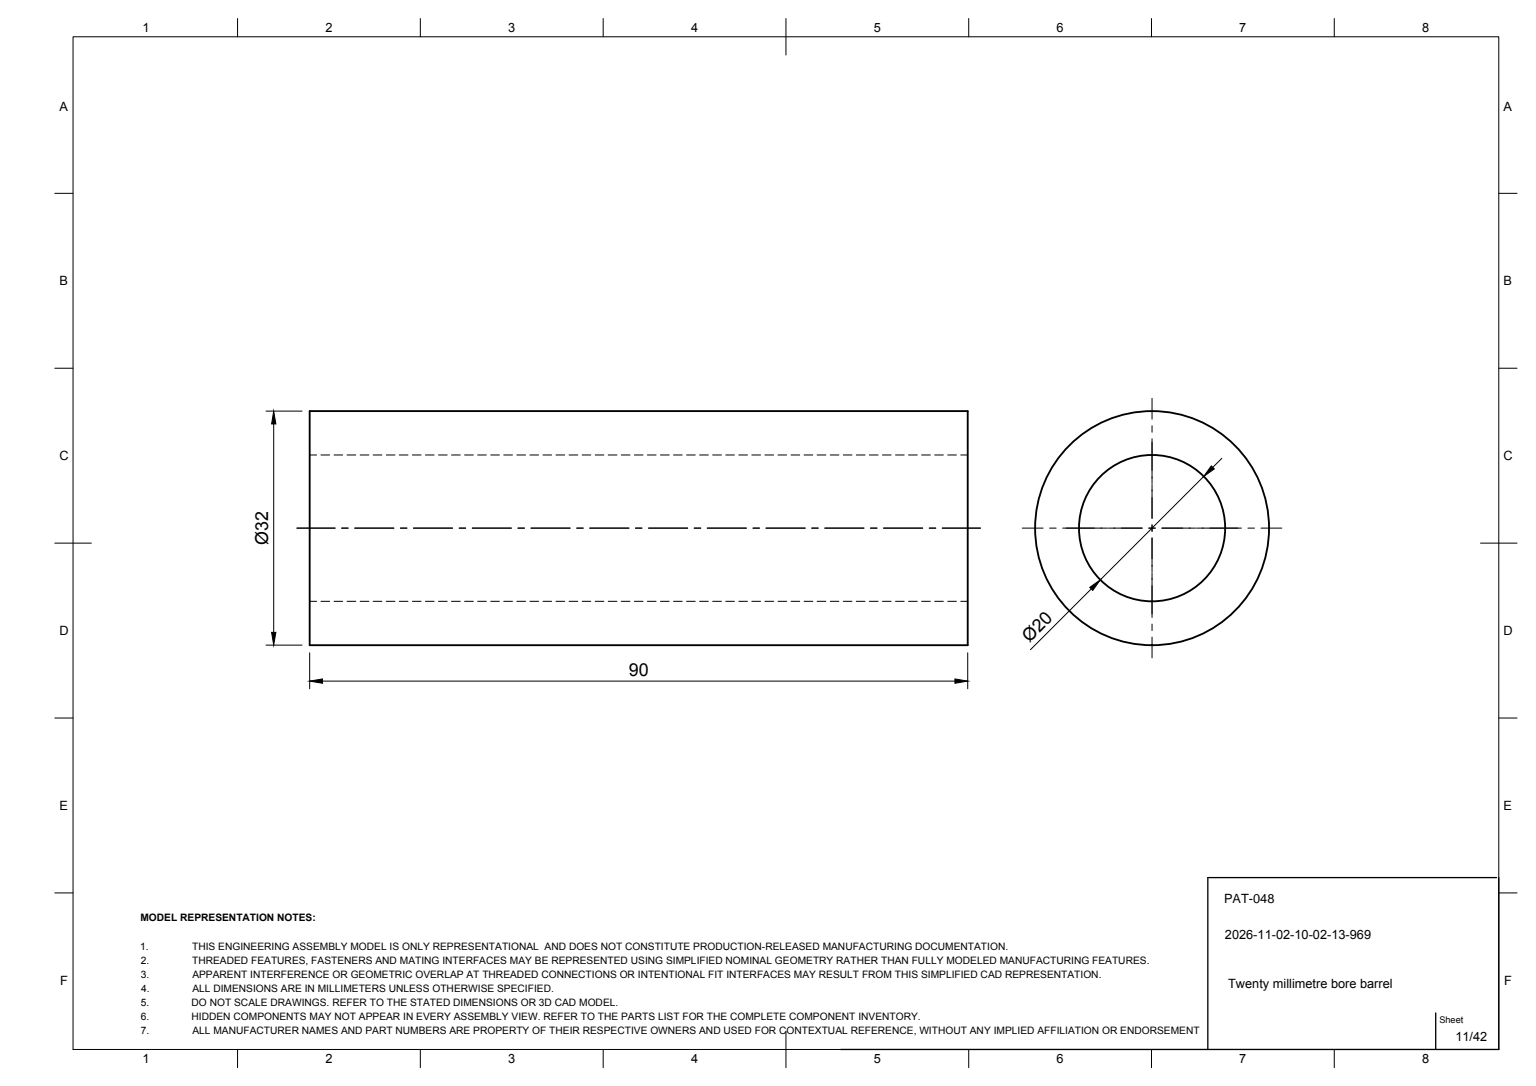
ISO-10303-21;
HEADER;
/* Generated by software containing ST-Developer
 * from STEP Tools, Inc. (www.steptools.com) 
 */

FILE_DESCRIPTION(
/* description */ ('Guided pneumatic stop gate'),
/* implementation_level */ '2;1');

FILE_NAME(
/* name */ 'Twenty millimetre bore barrel.step',
/* time_stamp */ '2026-10-27T21:43:45-07:00',
/* author */ (''),
/* organization */ (''),
/* preprocessor_version */ 'ST-DEVELOPER v20.2',
/* originating_system */ 'Autodesk Translation Framework v15.17.0.0',
/* authorisation */ '');

FILE_SCHEMA (('AUTOMOTIVE_DESIGN { 1 0 10303 214 3 1 1 }'));
ENDSEC;

DATA;
#10=MECHANICAL_DESIGN_GEOMETRIC_PRESENTATION_REPRESENTATION('',(#541),#14392);
#457=SHAPE_REPRESENTATION_RELATIONSHIP('SRR','None',#14591,#499);
#499=ADVANCED_BREP_SHAPE_REPRESENTATION('',(#583),#14353);
#541=STYLED_ITEM('',(#14884),#583);
#583=MANIFOLD_SOLID_BREP('Body1',#7881);
#663=FACE_BOUND('',#1777,.T.);
#664=FACE_BOUND('',#1779,.T.);
#921=PLANE('',#8642);
#922=PLANE('',#8643);
#1251=FACE_OUTER_BOUND('',#1774,.T.);
#1252=FACE_OUTER_BOUND('',#1775,.T.);
#1253=FACE_OUTER_BOUND('',#1776,.T.);
#1254=FACE_OUTER_BOUND('',#1778,.T.);
#1774=EDGE_LOOP('',(#5862,#5863,#5864,#5865));
#1775=EDGE_LOOP('',(#5866,#5867,#5868,#5869));
#1776=EDGE_LOOP('',(#5870));
#1777=EDGE_LOOP('',(#5871));
#1778=EDGE_LOOP('',(#5872));
#1779=EDGE_LOOP('',(#5873));
#2441=LINE('',#12509,#2986);
#2442=LINE('',#12515,#2987);
#2986=VECTOR('',#10052,1.);
#2987=VECTOR('',#10059,1.6);
#3464=CIRCLE('',#8637,1.);
#3465=CIRCLE('',#8638,1.);
#3466=CIRCLE('',#8640,1.6);
#3467=CIRCLE('',#8641,1.6);
#3907=VERTEX_POINT('',#12506);
#3908=VERTEX_POINT('',#12508);
#3909=VERTEX_POINT('',#12512);
#3910=VERTEX_POINT('',#12514);
#4629=EDGE_CURVE('',#3907,#3907,#3464,.T.);
#4630=EDGE_CURVE('',#3907,#3908,#2441,.T.);
#4631=EDGE_CURVE('',#3908,#3908,#3465,.T.);
#4632=EDGE_CURVE('',#3909,#3909,#3466,.T.);
#4633=EDGE_CURVE('',#3909,#3910,#2442,.T.);
#4634=EDGE_CURVE('',#3910,#3910,#3467,.T.);
#5862=ORIENTED_EDGE('',*,*,#4629,.F.);
#5863=ORIENTED_EDGE('',*,*,#4630,.T.);
#5864=ORIENTED_EDGE('',*,*,#4631,.T.);
#5865=ORIENTED_EDGE('',*,*,#4630,.F.);
#5866=ORIENTED_EDGE('',*,*,#4632,.F.);
#5867=ORIENTED_EDGE('',*,*,#4633,.T.);
#5868=ORIENTED_EDGE('',*,*,#4634,.T.);
#5869=ORIENTED_EDGE('',*,*,#4633,.F.);
#5870=ORIENTED_EDGE('',*,*,#4632,.T.);
#5871=ORIENTED_EDGE('',*,*,#4629,.T.);
#5872=ORIENTED_EDGE('',*,*,#4634,.F.);
#5873=ORIENTED_EDGE('',*,*,#4631,.F.);
#7283=CYLINDRICAL_SURFACE('',#8636,1.);
#7284=CYLINDRICAL_SURFACE('',#8639,1.6);
#7533=ADVANCED_FACE('',(#1251),#7283,.F.);
#7534=ADVANCED_FACE('',(#1252),#7284,.T.);
#7535=ADVANCED_FACE('',(#1253,#663),#921,.T.);
#7536=ADVANCED_FACE('',(#1254,#664),#922,.F.);
#7881=CLOSED_SHELL('',(#7533,#7534,#7535,#7536));
#8635=AXIS2_PLACEMENT_3D('',#12504,#10046,#10047);
#8636=AXIS2_PLACEMENT_3D('',#12505,#10048,#10049);
#8637=AXIS2_PLACEMENT_3D('',#12507,#10050,#10051);
#8638=AXIS2_PLACEMENT_3D('',#12510,#10053,#10054);
#8639=AXIS2_PLACEMENT_3D('',#12511,#10055,#10056);
#8640=AXIS2_PLACEMENT_3D('',#12513,#10057,#10058);
#8641=AXIS2_PLACEMENT_3D('',#12516,#10060,#10061);
#8642=AXIS2_PLACEMENT_3D('',#12517,#10062,#10063);
#8643=AXIS2_PLACEMENT_3D('',#12518,#10064,#10065);
#10046=DIRECTION('axis',(0.,0.,1.));
#10047=DIRECTION('refdir',(1.,0.,0.));
#10048=DIRECTION('center_axis',(0.,1.,0.));
#10049=DIRECTION('ref_axis',(1.,0.,0.));
#10050=DIRECTION('center_axis',(0.,-1.,0.));
#10051=DIRECTION('ref_axis',(1.,0.,0.));
#10052=DIRECTION('',(0.,-1.,0.));
#10053=DIRECTION('center_axis',(0.,-1.,0.));
#10054=DIRECTION('ref_axis',(1.,0.,0.));
#10055=DIRECTION('center_axis',(0.,1.,0.));
#10056=DIRECTION('ref_axis',(1.,0.,0.));
#10057=DIRECTION('center_axis',(0.,1.,0.));
#10058=DIRECTION('ref_axis',(1.,0.,0.));
#10059=DIRECTION('',(0.,-1.,0.));
#10060=DIRECTION('center_axis',(0.,1.,0.));
#10061=DIRECTION('ref_axis',(1.,0.,0.));
#10062=DIRECTION('center_axis',(0.,1.,0.));
#10063=DIRECTION('ref_axis',(1.,0.,0.));
#10064=DIRECTION('center_axis',(0.,1.,0.));
#10065=DIRECTION('ref_axis',(1.,0.,0.));
#12504=CARTESIAN_POINT('',(0.,0.,0.));
#12505=CARTESIAN_POINT('Origin',(0.,1.8,4.5));
#12506=CARTESIAN_POINT('',(-1.,10.8,4.5));
#12507=CARTESIAN_POINT('Origin',(0.,10.8,4.5));
#12508=CARTESIAN_POINT('',(-1.,1.8,4.5));
#12509=CARTESIAN_POINT('',(-1.,1.8,4.5));
#12510=CARTESIAN_POINT('Origin',(0.,1.8,4.5));
#12511=CARTESIAN_POINT('Origin',(0.,1.8,4.5));
#12512=CARTESIAN_POINT('',(-1.6,10.8,4.5));
#12513=CARTESIAN_POINT('Origin',(0.,10.8,4.5));
#12514=CARTESIAN_POINT('',(-1.6,1.8,4.5));
#12515=CARTESIAN_POINT('',(-1.6,1.8,4.5));
#12516=CARTESIAN_POINT('Origin',(0.,1.8,4.5));
#12517=CARTESIAN_POINT('Origin',(0.,10.8,4.5));
#12518=CARTESIAN_POINT('Origin',(0.,1.8,4.5));
#14305=UNCERTAINTY_MEASURE_WITH_UNIT(LENGTH_MEASURE(0.001),#14393,
'DISTANCE_ACCURACY_VALUE',
'Maximum model space distance between geometric entities at asserted c
onnectivities');
#14344=UNCERTAINTY_MEASURE_WITH_UNIT(LENGTH_MEASURE(0.001),#14393,
'DISTANCE_ACCURACY_VALUE',
'Maximum model space distance between geometric entities at asserted c
onnectivities');
#14353=(
GEOMETRIC_REPRESENTATION_CONTEXT(3)
GLOBAL_UNCERTAINTY_ASSIGNED_CONTEXT((#14305))
GLOBAL_UNIT_ASSIGNED_CONTEXT((#14393,#14395,#14396))
REPRESENTATION_CONTEXT('','3D')
);
#14392=(
GEOMETRIC_REPRESENTATION_CONTEXT(3)
GLOBAL_UNCERTAINTY_ASSIGNED_CONTEXT((#14344))
GLOBAL_UNIT_ASSIGNED_CONTEXT((#14393,#14395,#14396))
REPRESENTATION_CONTEXT('','3D')
);
#14393=(
LENGTH_UNIT()
NAMED_UNIT(*)
SI_UNIT(.CENTI.,.METRE.)
);
#14395=(
NAMED_UNIT(*)
PLANE_ANGLE_UNIT()
SI_UNIT($,.RADIAN.)
);
#14396=(
NAMED_UNIT(*)
SI_UNIT($,.STERADIAN.)
SOLID_ANGLE_UNIT()
);
#14405=SHAPE_DEFINITION_REPRESENTATION(#14452,#14591);
#14452=PRODUCT_DEFINITION_SHAPE('',$,#14639);
#14591=SHAPE_REPRESENTATION('',(#8635),#14353);
#14630=PRODUCT_DEFINITION_CONTEXT('part definition',#14773,'design');
#14639=PRODUCT_DEFINITION('Twenty millimetre bore barrel',
'Twenty millimetre bore barrel',#14686,#14630);
#14686=PRODUCT_DEFINITION_FORMATION('',$,#14783);
#14773=APPLICATION_CONTEXT(
'Core Data for Automotive Mechanical Design Process');
#14774=PRODUCT_CONTEXT('part definition',#14773,'mechanical');
#14783=PRODUCT('Twenty millimetre bore barrel',
'Twenty millimetre bore barrel','Twenty millimetre bore barrel',(#14774));
#14878=COLOUR_RGB('Sky Blue',0.24,0.69,0.87);
#14879=FILL_AREA_STYLE_COLOUR('',#14878);
#14880=FILL_AREA_STYLE('',(#14879));
#14881=SURFACE_STYLE_FILL_AREA(#14880);
#14882=SURFACE_SIDE_STYLE('',(#14881));
#14883=SURFACE_STYLE_USAGE(.BOTH.,#14882);
#14884=PRESENTATION_STYLE_ASSIGNMENT((#14883));
ENDSEC;
END-ISO-10303-21;
